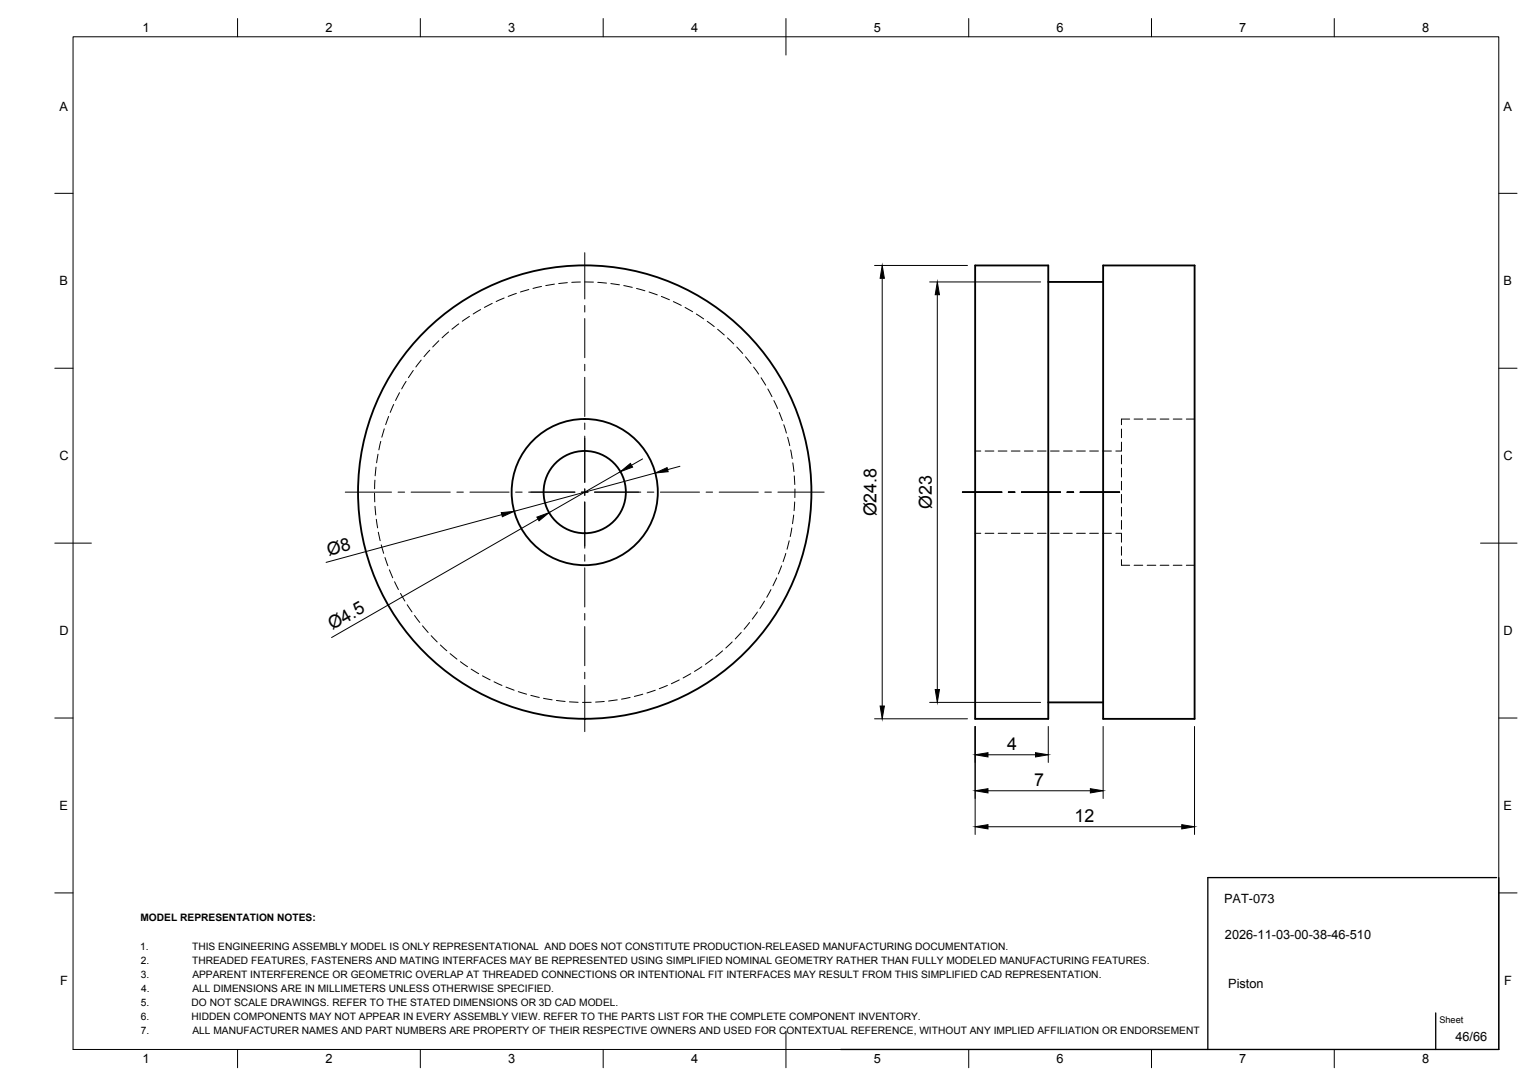
ISO-10303-21;
HEADER;
/* Generated by software containing ST-Developer
 * from STEP Tools, Inc. (www.steptools.com) 
 */

FILE_DESCRIPTION(
/* description */ ('Manual piston pump'),
/* implementation_level */ '2;1');

FILE_NAME(
/* name */ 'Piston.step',
/* time_stamp */ '2026-11-02T16:54:23-08:00',
/* author */ (''),
/* organization */ (''),
/* preprocessor_version */ 'ST-DEVELOPER v20.2',
/* originating_system */ 'Autodesk Translation Framework v15.17.0.0',
/* authorisation */ '');

FILE_SCHEMA (('AUTOMOTIVE_DESIGN { 1 0 10303 214 3 1 1 }'));
ENDSEC;

DATA;
#10=MECHANICAL_DESIGN_GEOMETRIC_PRESENTATION_REPRESENTATION('',(#737),#19043);
#603=SHAPE_REPRESENTATION_RELATIONSHIP('SRR','None',#19352,#666);
#666=ADVANCED_BREP_SHAPE_REPRESENTATION('',(#806),#19019);
#737=STYLED_ITEM('',(#19661),#806);
#806=MANIFOLD_SOLID_BREP('Body1',#9524);
#1000=FACE_BOUND('',#2454,.T.);
#1001=FACE_BOUND('',#2457,.T.);
#1002=FACE_BOUND('',#2459,.T.);
#1003=FACE_BOUND('',#2464,.T.);
#1004=FACE_BOUND('',#2466,.T.);
#1238=CYLINDRICAL_SURFACE('',#11077,0.4);
#1239=CYLINDRICAL_SURFACE('',#11082,1.15);
#1240=CYLINDRICAL_SURFACE('',#11089,1.24);
#1241=CYLINDRICAL_SURFACE('',#11091,0.225);
#1242=CYLINDRICAL_SURFACE('',#11093,1.24);
#1704=FACE_OUTER_BOUND('',#2452,.T.);
#1705=FACE_OUTER_BOUND('',#2453,.T.);
#1706=FACE_OUTER_BOUND('',#2455,.T.);
#1707=FACE_OUTER_BOUND('',#2456,.T.);
#1708=FACE_OUTER_BOUND('',#2458,.T.);
#1709=FACE_OUTER_BOUND('',#2460,.T.);
#1710=FACE_OUTER_BOUND('',#2461,.T.);
#1711=FACE_OUTER_BOUND('',#2462,.T.);
#1712=FACE_OUTER_BOUND('',#2463,.T.);
#1713=FACE_OUTER_BOUND('',#2465,.T.);
#2452=EDGE_LOOP('',(#7943,#7944,#7945,#7946));
#2453=EDGE_LOOP('',(#7947));
#2454=EDGE_LOOP('',(#7948));
#2455=EDGE_LOOP('',(#7949,#7950,#7951,#7952));
#2456=EDGE_LOOP('',(#7953));
#2457=EDGE_LOOP('',(#7954));
#2458=EDGE_LOOP('',(#7955));
#2459=EDGE_LOOP('',(#7956));
#2460=EDGE_LOOP('',(#7957,#7958,#7959,#7960));
#2461=EDGE_LOOP('',(#7961,#7962,#7963,#7964));
#2462=EDGE_LOOP('',(#7965,#7966,#7967,#7968));
#2463=EDGE_LOOP('',(#7969));
#2464=EDGE_LOOP('',(#7970));
#2465=EDGE_LOOP('',(#7971));
#2466=EDGE_LOOP('',(#7972));
#3026=CIRCLE('',#11078,0.4);
#3027=CIRCLE('',#11079,0.4);
#3028=CIRCLE('',#11081,0.225);
#3029=CIRCLE('',#11083,1.15);
#3030=CIRCLE('',#11084,1.15);
#3031=CIRCLE('',#11086,1.24);
#3032=CIRCLE('',#11088,1.24);
#3033=CIRCLE('',#11090,1.24);
#3034=CIRCLE('',#11092,0.225);
#3035=CIRCLE('',#11094,1.24);
#3573=LINE('',#17960,#4177);
#3574=LINE('',#17969,#4178);
#3575=LINE('',#17979,#4179);
#3576=LINE('',#17983,#4180);
#3577=LINE('',#17988,#4181);
#4177=VECTOR('',#13593,0.4);
#4178=VECTOR('',#13604,1.15);
#4179=VECTOR('',#13617,1.24);
#4180=VECTOR('',#13622,0.225);
#4181=VECTOR('',#13629,1.24);
#4917=VERTEX_POINT('',#17957);
#4918=VERTEX_POINT('',#17959);
#4919=VERTEX_POINT('',#17963);
#4920=VERTEX_POINT('',#17966);
#4921=VERTEX_POINT('',#17968);
#4922=VERTEX_POINT('',#17972);
#4923=VERTEX_POINT('',#17975);
#4924=VERTEX_POINT('',#17978);
#4925=VERTEX_POINT('',#17982);
#4926=VERTEX_POINT('',#17986);
#5958=EDGE_CURVE('',#4917,#4917,#3026,.T.);
#5959=EDGE_CURVE('',#4917,#4918,#3573,.T.);
#5960=EDGE_CURVE('',#4918,#4918,#3027,.T.);
#5961=EDGE_CURVE('',#4919,#4919,#3028,.T.);
#5962=EDGE_CURVE('',#4920,#4920,#3029,.T.);
#5963=EDGE_CURVE('',#4920,#4921,#3574,.T.);
#5964=EDGE_CURVE('',#4921,#4921,#3030,.T.);
#5965=EDGE_CURVE('',#4922,#4922,#3031,.T.);
#5966=EDGE_CURVE('',#4923,#4923,#3032,.T.);
#5967=EDGE_CURVE('',#4923,#4924,#3575,.T.);
#5968=EDGE_CURVE('',#4924,#4924,#3033,.T.);
#5969=EDGE_CURVE('',#4919,#4925,#3576,.T.);
#5970=EDGE_CURVE('',#4925,#4925,#3034,.T.);
#5971=EDGE_CURVE('',#4926,#4926,#3035,.T.);
#5972=EDGE_CURVE('',#4926,#4922,#3577,.T.);
#7943=ORIENTED_EDGE('',*,*,#5958,.F.);
#7944=ORIENTED_EDGE('',*,*,#5959,.T.);
#7945=ORIENTED_EDGE('',*,*,#5960,.F.);
#7946=ORIENTED_EDGE('',*,*,#5959,.F.);
#7947=ORIENTED_EDGE('',*,*,#5958,.T.);
#7948=ORIENTED_EDGE('',*,*,#5961,.F.);
#7949=ORIENTED_EDGE('',*,*,#5962,.F.);
#7950=ORIENTED_EDGE('',*,*,#5963,.T.);
#7951=ORIENTED_EDGE('',*,*,#5964,.T.);
#7952=ORIENTED_EDGE('',*,*,#5963,.F.);
#7953=ORIENTED_EDGE('',*,*,#5965,.F.);
#7954=ORIENTED_EDGE('',*,*,#5964,.F.);
#7955=ORIENTED_EDGE('',*,*,#5966,.F.);
#7956=ORIENTED_EDGE('',*,*,#5962,.T.);
#7957=ORIENTED_EDGE('',*,*,#5966,.T.);
#7958=ORIENTED_EDGE('',*,*,#5967,.T.);
#7959=ORIENTED_EDGE('',*,*,#5968,.T.);
#7960=ORIENTED_EDGE('',*,*,#5967,.F.);
#7961=ORIENTED_EDGE('',*,*,#5961,.T.);
#7962=ORIENTED_EDGE('',*,*,#5969,.T.);
#7963=ORIENTED_EDGE('',*,*,#5970,.T.);
#7964=ORIENTED_EDGE('',*,*,#5969,.F.);
#7965=ORIENTED_EDGE('',*,*,#5971,.F.);
#7966=ORIENTED_EDGE('',*,*,#5972,.T.);
#7967=ORIENTED_EDGE('',*,*,#5965,.T.);
#7968=ORIENTED_EDGE('',*,*,#5972,.F.);
#7969=ORIENTED_EDGE('',*,*,#5971,.T.);
#7970=ORIENTED_EDGE('',*,*,#5960,.T.);
#7971=ORIENTED_EDGE('',*,*,#5968,.F.);
#7972=ORIENTED_EDGE('',*,*,#5970,.F.);
#8798=PLANE('',#11080);
#8799=PLANE('',#11085);
#8800=PLANE('',#11087);
#8801=PLANE('',#11095);
#8802=PLANE('',#11096);
#9309=ADVANCED_FACE('',(#1704),#1238,.F.);
#9310=ADVANCED_FACE('',(#1705,#1000),#8798,.T.);
#9311=ADVANCED_FACE('',(#1706),#1239,.T.);
#9312=ADVANCED_FACE('',(#1707,#1001),#8799,.F.);
#9313=ADVANCED_FACE('',(#1708,#1002),#8800,.T.);
#9314=ADVANCED_FACE('',(#1709),#1240,.T.);
#9315=ADVANCED_FACE('',(#1710),#1241,.F.);
#9316=ADVANCED_FACE('',(#1711),#1242,.T.);
#9317=ADVANCED_FACE('',(#1712,#1003),#8801,.T.);
#9318=ADVANCED_FACE('',(#1713,#1004),#8802,.F.);
#9524=CLOSED_SHELL('',(#9309,#9310,#9311,#9312,#9313,#9314,#9315,#9316,
#9317,#9318));
#11076=AXIS2_PLACEMENT_3D('',#17955,#13587,#13588);
#11077=AXIS2_PLACEMENT_3D('',#17956,#13589,#13590);
#11078=AXIS2_PLACEMENT_3D('',#17958,#13591,#13592);
#11079=AXIS2_PLACEMENT_3D('',#17961,#13594,#13595);
#11080=AXIS2_PLACEMENT_3D('',#17962,#13596,#13597);
#11081=AXIS2_PLACEMENT_3D('',#17964,#13598,#13599);
#11082=AXIS2_PLACEMENT_3D('',#17965,#13600,#13601);
#11083=AXIS2_PLACEMENT_3D('',#17967,#13602,#13603);
#11084=AXIS2_PLACEMENT_3D('',#17970,#13605,#13606);
#11085=AXIS2_PLACEMENT_3D('',#17971,#13607,#13608);
#11086=AXIS2_PLACEMENT_3D('',#17973,#13609,#13610);
#11087=AXIS2_PLACEMENT_3D('',#17974,#13611,#13612);
#11088=AXIS2_PLACEMENT_3D('',#17976,#13613,#13614);
#11089=AXIS2_PLACEMENT_3D('',#17977,#13615,#13616);
#11090=AXIS2_PLACEMENT_3D('',#17980,#13618,#13619);
#11091=AXIS2_PLACEMENT_3D('',#17981,#13620,#13621);
#11092=AXIS2_PLACEMENT_3D('',#17984,#13623,#13624);
#11093=AXIS2_PLACEMENT_3D('',#17985,#13625,#13626);
#11094=AXIS2_PLACEMENT_3D('',#17987,#13627,#13628);
#11095=AXIS2_PLACEMENT_3D('',#17989,#13630,#13631);
#11096=AXIS2_PLACEMENT_3D('',#17990,#13632,#13633);
#13587=DIRECTION('axis',(0.,0.,1.));
#13588=DIRECTION('refdir',(1.,0.,0.));
#13589=DIRECTION('center_axis',(0.,1.,0.));
#13590=DIRECTION('ref_axis',(1.,0.,0.));
#13591=DIRECTION('center_axis',(0.,1.,0.));
#13592=DIRECTION('ref_axis',(1.,0.,0.));
#13593=DIRECTION('',(0.,1.,0.));
#13594=DIRECTION('center_axis',(0.,-1.,0.));
#13595=DIRECTION('ref_axis',(1.,0.,0.));
#13596=DIRECTION('center_axis',(0.,1.,0.));
#13597=DIRECTION('ref_axis',(1.,0.,0.));
#13598=DIRECTION('center_axis',(0.,1.,0.));
#13599=DIRECTION('ref_axis',(1.,0.,0.));
#13600=DIRECTION('center_axis',(0.,1.,0.));
#13601=DIRECTION('ref_axis',(1.,0.,0.));
#13602=DIRECTION('center_axis',(0.,-1.,0.));
#13603=DIRECTION('ref_axis',(1.,0.,0.));
#13604=DIRECTION('',(0.,1.,0.));
#13605=DIRECTION('center_axis',(0.,-1.,0.));
#13606=DIRECTION('ref_axis',(1.,0.,0.));
#13607=DIRECTION('center_axis',(0.,1.,0.));
#13608=DIRECTION('ref_axis',(1.,0.,0.));
#13609=DIRECTION('center_axis',(0.,1.,0.));
#13610=DIRECTION('ref_axis',(1.,0.,0.));
#13611=DIRECTION('center_axis',(0.,1.,0.));
#13612=DIRECTION('ref_axis',(1.,0.,0.));
#13613=DIRECTION('center_axis',(0.,-1.,0.));
#13614=DIRECTION('ref_axis',(1.,0.,0.));
#13615=DIRECTION('center_axis',(0.,1.,0.));
#13616=DIRECTION('ref_axis',(1.,0.,0.));
#13617=DIRECTION('',(0.,-1.,0.));
#13618=DIRECTION('center_axis',(0.,1.,0.));
#13619=DIRECTION('ref_axis',(1.,0.,0.));
#13620=DIRECTION('center_axis',(0.,1.,0.));
#13621=DIRECTION('ref_axis',(1.,0.,0.));
#13622=DIRECTION('',(0.,-1.,0.));
#13623=DIRECTION('center_axis',(0.,-1.,0.));
#13624=DIRECTION('ref_axis',(1.,0.,0.));
#13625=DIRECTION('center_axis',(0.,1.,0.));
#13626=DIRECTION('ref_axis',(1.,0.,0.));
#13627=DIRECTION('center_axis',(0.,1.,0.));
#13628=DIRECTION('ref_axis',(1.,0.,0.));
#13629=DIRECTION('',(0.,-1.,0.));
#13630=DIRECTION('center_axis',(0.,1.,0.));
#13631=DIRECTION('ref_axis',(1.,0.,0.));
#13632=DIRECTION('center_axis',(0.,1.,0.));
#13633=DIRECTION('ref_axis',(1.,0.,0.));
#17955=CARTESIAN_POINT('',(0.,0.,0.));
#17956=CARTESIAN_POINT('Origin',(0.,3.2,4.5));
#17957=CARTESIAN_POINT('',(-0.4,3.2,4.5));
#17958=CARTESIAN_POINT('Origin',(0.,3.2,4.5));
#17959=CARTESIAN_POINT('',(-0.4,3.6,4.5));
#17960=CARTESIAN_POINT('',(-0.4,3.2,4.5));
#17961=CARTESIAN_POINT('Origin',(0.,3.6,4.5));
#17962=CARTESIAN_POINT('Origin',(0.,3.2,4.5));
#17963=CARTESIAN_POINT('',(-0.225,3.2,4.5));
#17964=CARTESIAN_POINT('Origin',(0.,3.2,4.5));
#17965=CARTESIAN_POINT('Origin',(0.,2.8,4.5));
#17966=CARTESIAN_POINT('',(-1.15,2.8,4.5));
#17967=CARTESIAN_POINT('Origin',(0.,2.8,4.5));
#17968=CARTESIAN_POINT('',(-1.15,3.1,4.5));
#17969=CARTESIAN_POINT('',(-1.15,2.8,4.5));
#17970=CARTESIAN_POINT('Origin',(0.,3.1,4.5));
#17971=CARTESIAN_POINT('Origin',(0.,3.1,4.5));
#17972=CARTESIAN_POINT('',(-1.24,3.1,4.5));
#17973=CARTESIAN_POINT('Origin',(0.,3.1,4.5));
#17974=CARTESIAN_POINT('Origin',(0.,2.8,4.5));
#17975=CARTESIAN_POINT('',(-1.24,2.8,4.5));
#17976=CARTESIAN_POINT('Origin',(0.,2.8,4.5));
#17977=CARTESIAN_POINT('Origin',(0.,2.4,4.5));
#17978=CARTESIAN_POINT('',(-1.24,2.4,4.5));
#17979=CARTESIAN_POINT('',(-1.24,2.4,4.5));
#17980=CARTESIAN_POINT('Origin',(0.,2.4,4.5));
#17981=CARTESIAN_POINT('Origin',(0.,2.4,4.5));
#17982=CARTESIAN_POINT('',(-0.225,2.4,4.5));
#17983=CARTESIAN_POINT('',(-0.225,2.4,4.5));
#17984=CARTESIAN_POINT('Origin',(0.,2.4,4.5));
#17985=CARTESIAN_POINT('Origin',(0.,2.4,4.5));
#17986=CARTESIAN_POINT('',(-1.24,3.6,4.5));
#17987=CARTESIAN_POINT('Origin',(0.,3.6,4.5));
#17988=CARTESIAN_POINT('',(-1.24,2.4,4.5));
#17989=CARTESIAN_POINT('Origin',(0.,3.6,4.5));
#17990=CARTESIAN_POINT('Origin',(0.,2.4,4.5));
#18948=UNCERTAINTY_MEASURE_WITH_UNIT(LENGTH_MEASURE(0.001),#19044,
'DISTANCE_ACCURACY_VALUE',
'Maximum model space distance between geometric entities at asserted c
onnectivities');
#18972=UNCERTAINTY_MEASURE_WITH_UNIT(LENGTH_MEASURE(0.001),#19044,
'DISTANCE_ACCURACY_VALUE',
'Maximum model space distance between geometric entities at asserted c
onnectivities');
#19019=(
GEOMETRIC_REPRESENTATION_CONTEXT(3)
GLOBAL_UNCERTAINTY_ASSIGNED_CONTEXT((#18948))
GLOBAL_UNIT_ASSIGNED_CONTEXT((#19044,#19046,#19047))
REPRESENTATION_CONTEXT('','3D')
);
#19043=(
GEOMETRIC_REPRESENTATION_CONTEXT(3)
GLOBAL_UNCERTAINTY_ASSIGNED_CONTEXT((#18972))
GLOBAL_UNIT_ASSIGNED_CONTEXT((#19044,#19046,#19047))
REPRESENTATION_CONTEXT('','3D')
);
#19044=(
LENGTH_UNIT()
NAMED_UNIT(*)
SI_UNIT(.CENTI.,.METRE.)
);
#19046=(
NAMED_UNIT(*)
PLANE_ANGLE_UNIT()
SI_UNIT($,.RADIAN.)
);
#19047=(
NAMED_UNIT(*)
SI_UNIT($,.STERADIAN.)
SOLID_ANGLE_UNIT()
);
#19094=SHAPE_DEFINITION_REPRESENTATION(#19171,#19352);
#19171=PRODUCT_DEFINITION_SHAPE('',$,#19423);
#19352=SHAPE_REPRESENTATION('',(#11076),#19019);
#19376=PRODUCT_DEFINITION_CONTEXT('part definition',#19588,'design');
#19423=PRODUCT_DEFINITION('2026-11-03-00-38-46-510','Piston',#19493,#19376);
#19493=PRODUCT_DEFINITION_FORMATION('',$,#19636);
#19588=APPLICATION_CONTEXT(
'Core Data for Automotive Mechanical Design Process');
#19589=PRODUCT_CONTEXT('part definition',#19588,'mechanical');
#19636=PRODUCT('2026-11-03-00-38-46-510','Piston','Piston',(#19589));
#19661=PRESENTATION_STYLE_ASSIGNMENT((#19667));
#19667=SURFACE_STYLE_USAGE(.BOTH.,#19673);
#19673=SURFACE_SIDE_STYLE('',(#19679));
#19679=SURFACE_STYLE_FILL_AREA(#19685);
#19685=FILL_AREA_STYLE('CAD Library Painted - Engineering blue',(#19691));
#19691=FILL_AREA_STYLE_COLOUR('CAD Library Painted - Engineering blue',
#19697);
#19697=COLOUR_RGB('CAD Library Painted - Engineering blue',0.12156862745098,
0.356862745098039,0.6);
ENDSEC;
END-ISO-10303-21;
